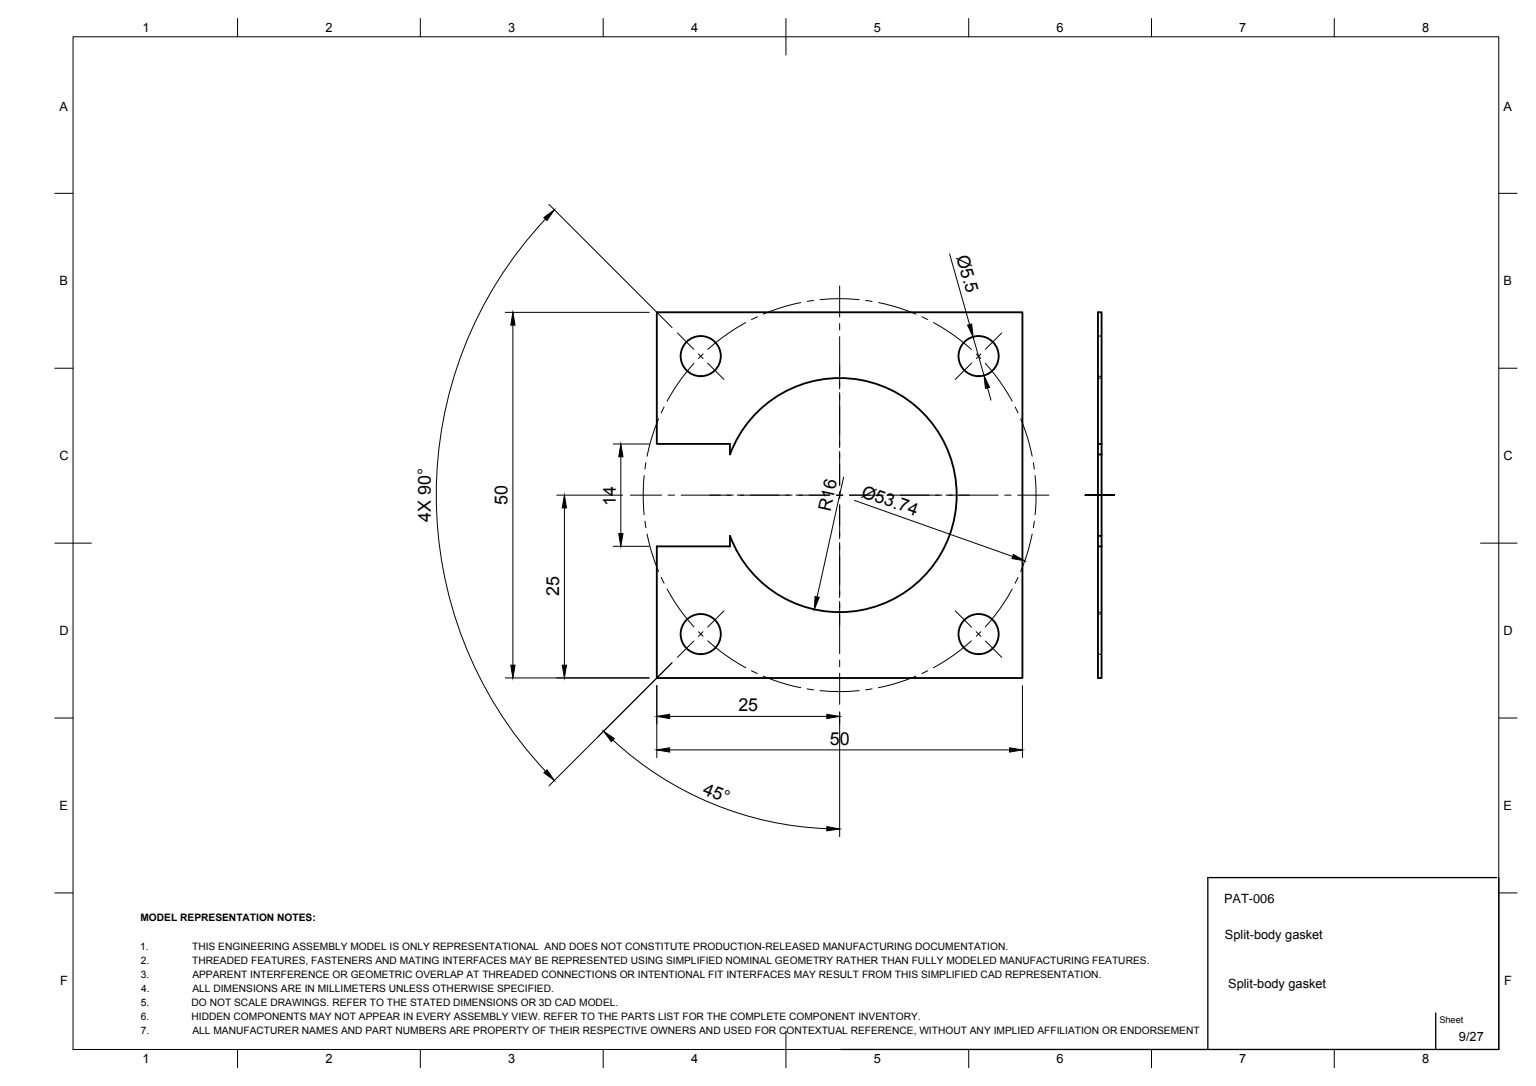
ISO-10303-21;
HEADER;
/* Generated by software containing ST-Developer
 * from STEP Tools, Inc. (www.steptools.com) 
 */

FILE_DESCRIPTION(
/* description */ ('Ball-type isolation valve (generic)'),
/* implementation_level */ '2;1');

FILE_NAME(
/* name */ 'Split-body gasket.step',
/* time_stamp */ '2026-10-27T10:53:05-07:00',
/* author */ (''),
/* organization */ (''),
/* preprocessor_version */ 'ST-DEVELOPER v20.2',
/* originating_system */ 'Autodesk Translation Framework v15.17.0.0',
/* authorisation */ '');

FILE_SCHEMA (('AUTOMOTIVE_DESIGN { 1 0 10303 214 3 1 1 }'));
ENDSEC;

DATA;
#10=MECHANICAL_DESIGN_GEOMETRIC_PRESENTATION_REPRESENTATION('',(#281),#7425);
#229=SHAPE_REPRESENTATION_RELATIONSHIP('SRR','None',#7539,#255);
#255=ADVANCED_BREP_SHAPE_REPRESENTATION('',(#307),#7402);
#281=STYLED_ITEM('',(#7723),#307);
#307=MANIFOLD_SOLID_BREP('Body1',#4086);
#365=FACE_BOUND('',#923,.T.);
#366=FACE_BOUND('',#924,.T.);
#367=FACE_BOUND('',#925,.T.);
#368=FACE_BOUND('',#926,.T.);
#369=FACE_BOUND('',#934,.T.);
#370=FACE_BOUND('',#935,.T.);
#371=FACE_BOUND('',#936,.T.);
#372=FACE_BOUND('',#937,.T.);
#445=PLANE('',#4521);
#446=PLANE('',#4522);
#447=PLANE('',#4523);
#448=PLANE('',#4524);
#449=PLANE('',#4525);
#450=PLANE('',#4527);
#451=PLANE('',#4528);
#452=PLANE('',#4531);
#453=PLANE('',#4532);
#454=PLANE('',#4533);
#455=PLANE('',#4534);
#631=FACE_OUTER_BOUND('',#914,.T.);
#632=FACE_OUTER_BOUND('',#915,.T.);
#633=FACE_OUTER_BOUND('',#916,.T.);
#634=FACE_OUTER_BOUND('',#917,.T.);
#635=FACE_OUTER_BOUND('',#918,.T.);
#636=FACE_OUTER_BOUND('',#919,.T.);
#637=FACE_OUTER_BOUND('',#920,.T.);
#638=FACE_OUTER_BOUND('',#921,.T.);
#639=FACE_OUTER_BOUND('',#922,.T.);
#640=FACE_OUTER_BOUND('',#927,.T.);
#641=FACE_OUTER_BOUND('',#928,.T.);
#642=FACE_OUTER_BOUND('',#929,.T.);
#643=FACE_OUTER_BOUND('',#930,.T.);
#644=FACE_OUTER_BOUND('',#931,.T.);
#645=FACE_OUTER_BOUND('',#932,.T.);
#646=FACE_OUTER_BOUND('',#933,.T.);
#914=EDGE_LOOP('',(#2987,#2988,#2989,#2990));
#915=EDGE_LOOP('',(#2991,#2992,#2993,#2994));
#916=EDGE_LOOP('',(#2995,#2996,#2997,#2998));
#917=EDGE_LOOP('',(#2999,#3000,#3001,#3002));
#918=EDGE_LOOP('',(#3003,#3004,#3005,#3006));
#919=EDGE_LOOP('',(#3007,#3008,#3009,#3010));
#920=EDGE_LOOP('',(#3011,#3012,#3013,#3014));
#921=EDGE_LOOP('',(#3015,#3016,#3017,#3018));
#922=EDGE_LOOP('',(#3019,#3020,#3021,#3022,#3023,#3024,#3025,#3026,#3027,
#3028));
#923=EDGE_LOOP('',(#3029));
#924=EDGE_LOOP('',(#3030));
#925=EDGE_LOOP('',(#3031));
#926=EDGE_LOOP('',(#3032));
#927=EDGE_LOOP('',(#3033,#3034,#3035,#3036));
#928=EDGE_LOOP('',(#3037,#3038,#3039,#3040));
#929=EDGE_LOOP('',(#3041,#3042,#3043,#3044));
#930=EDGE_LOOP('',(#3045,#3046,#3047,#3048));
#931=EDGE_LOOP('',(#3049,#3050,#3051,#3052));
#932=EDGE_LOOP('',(#3053,#3054,#3055,#3056));
#933=EDGE_LOOP('',(#3057,#3058,#3059,#3060,#3061,#3062,#3063,#3064,#3065,
#3066));
#934=EDGE_LOOP('',(#3067));
#935=EDGE_LOOP('',(#3068));
#936=EDGE_LOOP('',(#3069));
#937=EDGE_LOOP('',(#3070));
#1219=LINE('',#6441,#1527);
#1220=LINE('',#6447,#1528);
#1221=LINE('',#6453,#1529);
#1222=LINE('',#6459,#1530);
#1223=LINE('',#6464,#1531);
#1224=LINE('',#6466,#1532);
#1225=LINE('',#6468,#1533);
#1226=LINE('',#6469,#1534);
#1227=LINE('',#6473,#1535);
#1228=LINE('',#6475,#1536);
#1229=LINE('',#6477,#1537);
#1230=LINE('',#6478,#1538);
#1231=LINE('',#6481,#1539);
#1232=LINE('',#6483,#1540);
#1233=LINE('',#6484,#1541);
#1234=LINE('',#6487,#1542);
#1235=LINE('',#6489,#1543);
#1236=LINE('',#6490,#1544);
#1237=LINE('',#6494,#1545);
#1238=LINE('',#6496,#1546);
#1239=LINE('',#6498,#1547);
#1240=LINE('',#6500,#1548);
#1241=LINE('',#6501,#1549);
#1242=LINE('',#6504,#1550);
#1243=LINE('',#6505,#1551);
#1244=LINE('',#6508,#1552);
#1245=LINE('',#6509,#1553);
#1246=LINE('',#6514,#1554);
#1247=LINE('',#6515,#1555);
#1248=LINE('',#6518,#1556);
#1249=LINE('',#6519,#1557);
#1250=LINE('',#6521,#1558);
#1527=VECTOR('',#5176,0.275);
#1528=VECTOR('',#5183,0.275);
#1529=VECTOR('',#5190,0.275);
#1530=VECTOR('',#5197,0.275);
#1531=VECTOR('',#5202,1.);
#1532=VECTOR('',#5203,1.);
#1533=VECTOR('',#5204,1.);
#1534=VECTOR('',#5205,1.);
#1535=VECTOR('',#5208,1.);
#1536=VECTOR('',#5209,1.);
#1537=VECTOR('',#5210,1.);
#1538=VECTOR('',#5211,1.);
#1539=VECTOR('',#5214,1.);
#1540=VECTOR('',#5215,1.);
#1541=VECTOR('',#5216,1.);
#1542=VECTOR('',#5219,1.);
#1543=VECTOR('',#5220,1.);
#1544=VECTOR('',#5221,1.);
#1545=VECTOR('',#5226,1.);
#1546=VECTOR('',#5227,1.);
#1547=VECTOR('',#5228,1.);
#1548=VECTOR('',#5229,1.);
#1549=VECTOR('',#5230,1.);
#1550=VECTOR('',#5233,1.);
#1551=VECTOR('',#5234,1.);
#1552=VECTOR('',#5237,1.);
#1553=VECTOR('',#5238,1.);
#1554=VECTOR('',#5245,1.);
#1555=VECTOR('',#5246,1.);
#1556=VECTOR('',#5249,1.);
#1557=VECTOR('',#5250,1.);
#1558=VECTOR('',#5253,1.);
#1833=CIRCLE('',#4510,0.275);
#1834=CIRCLE('',#4511,0.275);
#1835=CIRCLE('',#4513,0.275);
#1836=CIRCLE('',#4514,0.275);
#1837=CIRCLE('',#4516,0.275);
#1838=CIRCLE('',#4517,0.275);
#1839=CIRCLE('',#4519,0.275);
#1840=CIRCLE('',#4520,0.275);
#1841=CIRCLE('',#4526,1.6);
#1842=CIRCLE('',#4530,1.6);
#2028=VERTEX_POINT('',#6438);
#2029=VERTEX_POINT('',#6440);
#2030=VERTEX_POINT('',#6444);
#2031=VERTEX_POINT('',#6446);
#2032=VERTEX_POINT('',#6450);
#2033=VERTEX_POINT('',#6452);
#2034=VERTEX_POINT('',#6456);
#2035=VERTEX_POINT('',#6458);
#2036=VERTEX_POINT('',#6462);
#2037=VERTEX_POINT('',#6463);
#2038=VERTEX_POINT('',#6465);
#2039=VERTEX_POINT('',#6467);
#2040=VERTEX_POINT('',#6471);
#2041=VERTEX_POINT('',#6472);
#2042=VERTEX_POINT('',#6474);
#2043=VERTEX_POINT('',#6476);
#2044=VERTEX_POINT('',#6480);
#2045=VERTEX_POINT('',#6482);
#2046=VERTEX_POINT('',#6486);
#2047=VERTEX_POINT('',#6488);
#2048=VERTEX_POINT('',#6493);
#2049=VERTEX_POINT('',#6495);
#2050=VERTEX_POINT('',#6497);
#2051=VERTEX_POINT('',#6499);
#2052=VERTEX_POINT('',#6503);
#2053=VERTEX_POINT('',#6507);
#2054=VERTEX_POINT('',#6513);
#2055=VERTEX_POINT('',#6517);
#2386=EDGE_CURVE('',#2028,#2028,#1833,.T.);
#2387=EDGE_CURVE('',#2028,#2029,#1219,.T.);
#2388=EDGE_CURVE('',#2029,#2029,#1834,.T.);
#2389=EDGE_CURVE('',#2030,#2030,#1835,.T.);
#2390=EDGE_CURVE('',#2030,#2031,#1220,.T.);
#2391=EDGE_CURVE('',#2031,#2031,#1836,.T.);
#2392=EDGE_CURVE('',#2032,#2032,#1837,.T.);
#2393=EDGE_CURVE('',#2032,#2033,#1221,.T.);
#2394=EDGE_CURVE('',#2033,#2033,#1838,.T.);
#2395=EDGE_CURVE('',#2034,#2034,#1839,.T.);
#2396=EDGE_CURVE('',#2034,#2035,#1222,.T.);
#2397=EDGE_CURVE('',#2035,#2035,#1840,.T.);
#2398=EDGE_CURVE('',#2036,#2037,#1223,.T.);
#2399=EDGE_CURVE('',#2036,#2038,#1224,.T.);
#2400=EDGE_CURVE('',#2039,#2038,#1225,.T.);
#2401=EDGE_CURVE('',#2037,#2039,#1226,.T.);
#2402=EDGE_CURVE('',#2040,#2041,#1227,.T.);
#2403=EDGE_CURVE('',#2040,#2042,#1228,.T.);
#2404=EDGE_CURVE('',#2043,#2042,#1229,.T.);
#2405=EDGE_CURVE('',#2041,#2043,#1230,.T.);
#2406=EDGE_CURVE('',#2044,#2036,#1231,.T.);
#2407=EDGE_CURVE('',#2045,#2044,#1232,.T.);
#2408=EDGE_CURVE('',#2038,#2045,#1233,.T.);
#2409=EDGE_CURVE('',#2046,#2040,#1234,.T.);
#2410=EDGE_CURVE('',#2047,#2046,#1235,.T.);
#2411=EDGE_CURVE('',#2042,#2047,#1236,.T.);
#2412=EDGE_CURVE('',#2045,#2043,#1841,.T.);
#2413=EDGE_CURVE('',#2047,#2048,#1237,.T.);
#2414=EDGE_CURVE('',#2048,#2049,#1238,.T.);
#2415=EDGE_CURVE('',#2049,#2050,#1239,.T.);
#2416=EDGE_CURVE('',#2050,#2051,#1240,.T.);
#2417=EDGE_CURVE('',#2051,#2039,#1241,.T.);
#2418=EDGE_CURVE('',#2052,#2046,#1242,.T.);
#2419=EDGE_CURVE('',#2052,#2048,#1243,.T.);
#2420=EDGE_CURVE('',#2053,#2051,#1244,.T.);
#2421=EDGE_CURVE('',#2037,#2053,#1245,.T.);
#2422=EDGE_CURVE('',#2041,#2044,#1842,.T.);
#2423=EDGE_CURVE('',#2053,#2054,#1246,.T.);
#2424=EDGE_CURVE('',#2054,#2050,#1247,.T.);
#2425=EDGE_CURVE('',#2054,#2055,#1248,.T.);
#2426=EDGE_CURVE('',#2055,#2049,#1249,.T.);
#2427=EDGE_CURVE('',#2055,#2052,#1250,.T.);
#2987=ORIENTED_EDGE('',*,*,#2386,.F.);
#2988=ORIENTED_EDGE('',*,*,#2387,.T.);
#2989=ORIENTED_EDGE('',*,*,#2388,.F.);
#2990=ORIENTED_EDGE('',*,*,#2387,.F.);
#2991=ORIENTED_EDGE('',*,*,#2389,.F.);
#2992=ORIENTED_EDGE('',*,*,#2390,.T.);
#2993=ORIENTED_EDGE('',*,*,#2391,.F.);
#2994=ORIENTED_EDGE('',*,*,#2390,.F.);
#2995=ORIENTED_EDGE('',*,*,#2392,.F.);
#2996=ORIENTED_EDGE('',*,*,#2393,.T.);
#2997=ORIENTED_EDGE('',*,*,#2394,.F.);
#2998=ORIENTED_EDGE('',*,*,#2393,.F.);
#2999=ORIENTED_EDGE('',*,*,#2395,.F.);
#3000=ORIENTED_EDGE('',*,*,#2396,.T.);
#3001=ORIENTED_EDGE('',*,*,#2397,.F.);
#3002=ORIENTED_EDGE('',*,*,#2396,.F.);
#3003=ORIENTED_EDGE('',*,*,#2398,.F.);
#3004=ORIENTED_EDGE('',*,*,#2399,.T.);
#3005=ORIENTED_EDGE('',*,*,#2400,.F.);
#3006=ORIENTED_EDGE('',*,*,#2401,.F.);
#3007=ORIENTED_EDGE('',*,*,#2402,.F.);
#3008=ORIENTED_EDGE('',*,*,#2403,.T.);
#3009=ORIENTED_EDGE('',*,*,#2404,.F.);
#3010=ORIENTED_EDGE('',*,*,#2405,.F.);
#3011=ORIENTED_EDGE('',*,*,#2406,.F.);
#3012=ORIENTED_EDGE('',*,*,#2407,.F.);
#3013=ORIENTED_EDGE('',*,*,#2408,.F.);
#3014=ORIENTED_EDGE('',*,*,#2399,.F.);
#3015=ORIENTED_EDGE('',*,*,#2409,.F.);
#3016=ORIENTED_EDGE('',*,*,#2410,.F.);
#3017=ORIENTED_EDGE('',*,*,#2411,.F.);
#3018=ORIENTED_EDGE('',*,*,#2403,.F.);
#3019=ORIENTED_EDGE('',*,*,#2400,.T.);
#3020=ORIENTED_EDGE('',*,*,#2408,.T.);
#3021=ORIENTED_EDGE('',*,*,#2412,.T.);
#3022=ORIENTED_EDGE('',*,*,#2404,.T.);
#3023=ORIENTED_EDGE('',*,*,#2411,.T.);
#3024=ORIENTED_EDGE('',*,*,#2413,.T.);
#3025=ORIENTED_EDGE('',*,*,#2414,.T.);
#3026=ORIENTED_EDGE('',*,*,#2415,.T.);
#3027=ORIENTED_EDGE('',*,*,#2416,.T.);
#3028=ORIENTED_EDGE('',*,*,#2417,.T.);
#3029=ORIENTED_EDGE('',*,*,#2388,.T.);
#3030=ORIENTED_EDGE('',*,*,#2391,.T.);
#3031=ORIENTED_EDGE('',*,*,#2394,.T.);
#3032=ORIENTED_EDGE('',*,*,#2397,.T.);
#3033=ORIENTED_EDGE('',*,*,#2410,.T.);
#3034=ORIENTED_EDGE('',*,*,#2418,.F.);
#3035=ORIENTED_EDGE('',*,*,#2419,.T.);
#3036=ORIENTED_EDGE('',*,*,#2413,.F.);
#3037=ORIENTED_EDGE('',*,*,#2401,.T.);
#3038=ORIENTED_EDGE('',*,*,#2417,.F.);
#3039=ORIENTED_EDGE('',*,*,#2420,.F.);
#3040=ORIENTED_EDGE('',*,*,#2421,.F.);
#3041=ORIENTED_EDGE('',*,*,#2407,.T.);
#3042=ORIENTED_EDGE('',*,*,#2422,.F.);
#3043=ORIENTED_EDGE('',*,*,#2405,.T.);
#3044=ORIENTED_EDGE('',*,*,#2412,.F.);
#3045=ORIENTED_EDGE('',*,*,#2423,.F.);
#3046=ORIENTED_EDGE('',*,*,#2420,.T.);
#3047=ORIENTED_EDGE('',*,*,#2416,.F.);
#3048=ORIENTED_EDGE('',*,*,#2424,.F.);
#3049=ORIENTED_EDGE('',*,*,#2425,.F.);
#3050=ORIENTED_EDGE('',*,*,#2424,.T.);
#3051=ORIENTED_EDGE('',*,*,#2415,.F.);
#3052=ORIENTED_EDGE('',*,*,#2426,.F.);
#3053=ORIENTED_EDGE('',*,*,#2427,.F.);
#3054=ORIENTED_EDGE('',*,*,#2426,.T.);
#3055=ORIENTED_EDGE('',*,*,#2414,.F.);
#3056=ORIENTED_EDGE('',*,*,#2419,.F.);
#3057=ORIENTED_EDGE('',*,*,#2398,.T.);
#3058=ORIENTED_EDGE('',*,*,#2421,.T.);
#3059=ORIENTED_EDGE('',*,*,#2423,.T.);
#3060=ORIENTED_EDGE('',*,*,#2425,.T.);
#3061=ORIENTED_EDGE('',*,*,#2427,.T.);
#3062=ORIENTED_EDGE('',*,*,#2418,.T.);
#3063=ORIENTED_EDGE('',*,*,#2409,.T.);
#3064=ORIENTED_EDGE('',*,*,#2402,.T.);
#3065=ORIENTED_EDGE('',*,*,#2422,.T.);
#3066=ORIENTED_EDGE('',*,*,#2406,.T.);
#3067=ORIENTED_EDGE('',*,*,#2386,.T.);
#3068=ORIENTED_EDGE('',*,*,#2389,.T.);
#3069=ORIENTED_EDGE('',*,*,#2392,.T.);
#3070=ORIENTED_EDGE('',*,*,#2395,.T.);
#3787=CYLINDRICAL_SURFACE('',#4509,0.275);
#3788=CYLINDRICAL_SURFACE('',#4512,0.275);
#3789=CYLINDRICAL_SURFACE('',#4515,0.275);
#3790=CYLINDRICAL_SURFACE('',#4518,0.275);
#3791=CYLINDRICAL_SURFACE('',#4529,1.6);
#3885=ADVANCED_FACE('',(#631),#3787,.F.);
#3886=ADVANCED_FACE('',(#632),#3788,.F.);
#3887=ADVANCED_FACE('',(#633),#3789,.F.);
#3888=ADVANCED_FACE('',(#634),#3790,.F.);
#3889=ADVANCED_FACE('',(#635),#445,.F.);
#3890=ADVANCED_FACE('',(#636),#446,.F.);
#3891=ADVANCED_FACE('',(#637),#447,.F.);
#3892=ADVANCED_FACE('',(#638),#448,.F.);
#3893=ADVANCED_FACE('',(#639,#365,#366,#367,#368),#449,.T.);
#3894=ADVANCED_FACE('',(#640),#450,.T.);
#3895=ADVANCED_FACE('',(#641),#451,.T.);
#3896=ADVANCED_FACE('',(#642),#3791,.F.);
#3897=ADVANCED_FACE('',(#643),#452,.T.);
#3898=ADVANCED_FACE('',(#644),#453,.T.);
#3899=ADVANCED_FACE('',(#645),#454,.T.);
#3900=ADVANCED_FACE('',(#646,#369,#370,#371,#372),#455,.F.);
#4086=CLOSED_SHELL('',(#3885,#3886,#3887,#3888,#3889,#3890,#3891,#3892,
#3893,#3894,#3895,#3896,#3897,#3898,#3899,#3900));
#4508=AXIS2_PLACEMENT_3D('',#6436,#5170,#5171);
#4509=AXIS2_PLACEMENT_3D('',#6437,#5172,#5173);
#4510=AXIS2_PLACEMENT_3D('',#6439,#5174,#5175);
#4511=AXIS2_PLACEMENT_3D('',#6442,#5177,#5178);
#4512=AXIS2_PLACEMENT_3D('',#6443,#5179,#5180);
#4513=AXIS2_PLACEMENT_3D('',#6445,#5181,#5182);
#4514=AXIS2_PLACEMENT_3D('',#6448,#5184,#5185);
#4515=AXIS2_PLACEMENT_3D('',#6449,#5186,#5187);
#4516=AXIS2_PLACEMENT_3D('',#6451,#5188,#5189);
#4517=AXIS2_PLACEMENT_3D('',#6454,#5191,#5192);
#4518=AXIS2_PLACEMENT_3D('',#6455,#5193,#5194);
#4519=AXIS2_PLACEMENT_3D('',#6457,#5195,#5196);
#4520=AXIS2_PLACEMENT_3D('',#6460,#5198,#5199);
#4521=AXIS2_PLACEMENT_3D('',#6461,#5200,#5201);
#4522=AXIS2_PLACEMENT_3D('',#6470,#5206,#5207);
#4523=AXIS2_PLACEMENT_3D('',#6479,#5212,#5213);
#4524=AXIS2_PLACEMENT_3D('',#6485,#5217,#5218);
#4525=AXIS2_PLACEMENT_3D('',#6491,#5222,#5223);
#4526=AXIS2_PLACEMENT_3D('',#6492,#5224,#5225);
#4527=AXIS2_PLACEMENT_3D('',#6502,#5231,#5232);
#4528=AXIS2_PLACEMENT_3D('',#6506,#5235,#5236);
#4529=AXIS2_PLACEMENT_3D('',#6510,#5239,#5240);
#4530=AXIS2_PLACEMENT_3D('',#6511,#5241,#5242);
#4531=AXIS2_PLACEMENT_3D('',#6512,#5243,#5244);
#4532=AXIS2_PLACEMENT_3D('',#6516,#5247,#5248);
#4533=AXIS2_PLACEMENT_3D('',#6520,#5251,#5252);
#4534=AXIS2_PLACEMENT_3D('',#6522,#5254,#5255);
#5170=DIRECTION('axis',(0.,0.,1.));
#5171=DIRECTION('refdir',(1.,0.,0.));
#5172=DIRECTION('center_axis',(0.,1.,0.));
#5173=DIRECTION('ref_axis',(1.,0.,0.));
#5174=DIRECTION('center_axis',(0.,1.,0.));
#5175=DIRECTION('ref_axis',(1.,0.,0.));
#5176=DIRECTION('',(0.,1.,0.));
#5177=DIRECTION('center_axis',(0.,-1.,0.));
#5178=DIRECTION('ref_axis',(1.,0.,0.));
#5179=DIRECTION('center_axis',(0.,1.,0.));
#5180=DIRECTION('ref_axis',(1.,0.,0.));
#5181=DIRECTION('center_axis',(0.,1.,0.));
#5182=DIRECTION('ref_axis',(1.,0.,0.));
#5183=DIRECTION('',(0.,1.,0.));
#5184=DIRECTION('center_axis',(0.,-1.,0.));
#5185=DIRECTION('ref_axis',(1.,0.,0.));
#5186=DIRECTION('center_axis',(0.,1.,0.));
#5187=DIRECTION('ref_axis',(1.,0.,0.));
#5188=DIRECTION('center_axis',(0.,1.,0.));
#5189=DIRECTION('ref_axis',(1.,0.,0.));
#5190=DIRECTION('',(0.,1.,0.));
#5191=DIRECTION('center_axis',(0.,-1.,0.));
#5192=DIRECTION('ref_axis',(1.,0.,0.));
#5193=DIRECTION('center_axis',(0.,1.,0.));
#5194=DIRECTION('ref_axis',(1.,0.,0.));
#5195=DIRECTION('center_axis',(0.,1.,0.));
#5196=DIRECTION('ref_axis',(1.,0.,0.));
#5197=DIRECTION('',(0.,1.,0.));
#5198=DIRECTION('center_axis',(0.,-1.,0.));
#5199=DIRECTION('ref_axis',(1.,0.,0.));
#5200=DIRECTION('center_axis',(-1.,0.,0.));
#5201=DIRECTION('ref_axis',(0.,0.,1.));
#5202=DIRECTION('',(0.,0.,1.));
#5203=DIRECTION('',(0.,1.,0.));
#5204=DIRECTION('',(0.,0.,-1.));
#5205=DIRECTION('',(0.,1.,0.));
#5206=DIRECTION('center_axis',(0.,0.,-1.));
#5207=DIRECTION('ref_axis',(-1.,0.,0.));
#5208=DIRECTION('',(-1.,0.,0.));
#5209=DIRECTION('',(0.,1.,0.));
#5210=DIRECTION('',(1.,0.,0.));
#5211=DIRECTION('',(0.,1.,0.));
#5212=DIRECTION('center_axis',(0.,0.,-1.));
#5213=DIRECTION('ref_axis',(-1.,0.,0.));
#5214=DIRECTION('',(-1.,0.,0.));
#5215=DIRECTION('',(0.,-1.,0.));
#5216=DIRECTION('',(1.,0.,0.));
#5217=DIRECTION('center_axis',(1.,0.,0.));
#5218=DIRECTION('ref_axis',(0.,0.,-1.));
#5219=DIRECTION('',(0.,0.,-1.));
#5220=DIRECTION('',(0.,-1.,0.));
#5221=DIRECTION('',(0.,0.,1.));
#5222=DIRECTION('center_axis',(0.,1.,0.));
#5223=DIRECTION('ref_axis',(0.,0.,1.));
#5224=DIRECTION('center_axis',(0.,-1.,0.));
#5225=DIRECTION('ref_axis',(1.,0.,0.));
#5226=DIRECTION('',(1.,0.,0.));
#5227=DIRECTION('',(0.,0.,-1.));
#5228=DIRECTION('',(-1.,0.,0.));
#5229=DIRECTION('',(0.,0.,1.));
#5230=DIRECTION('',(1.,0.,0.));
#5231=DIRECTION('center_axis',(0.,0.,1.));
#5232=DIRECTION('ref_axis',(1.,0.,0.));
#5233=DIRECTION('',(-1.,0.,0.));
#5234=DIRECTION('',(0.,1.,0.));
#5235=DIRECTION('center_axis',(0.,0.,1.));
#5236=DIRECTION('ref_axis',(1.,0.,0.));
#5237=DIRECTION('',(0.,1.,0.));
#5238=DIRECTION('',(-1.,0.,0.));
#5239=DIRECTION('center_axis',(0.,1.,0.));
#5240=DIRECTION('ref_axis',(-1.83697019872103E-16,0.,-1.));
#5241=DIRECTION('center_axis',(0.,1.,0.));
#5242=DIRECTION('ref_axis',(1.,0.,0.));
#5243=DIRECTION('center_axis',(-1.,0.,0.));
#5244=DIRECTION('ref_axis',(0.,0.,1.));
#5245=DIRECTION('',(0.,0.,-1.));
#5246=DIRECTION('',(0.,1.,0.));
#5247=DIRECTION('center_axis',(0.,0.,-1.));
#5248=DIRECTION('ref_axis',(-1.,0.,0.));
#5249=DIRECTION('',(1.,0.,0.));
#5250=DIRECTION('',(0.,1.,0.));
#5251=DIRECTION('center_axis',(1.,0.,0.));
#5252=DIRECTION('ref_axis',(0.,0.,-1.));
#5253=DIRECTION('',(0.,0.,1.));
#5254=DIRECTION('center_axis',(0.,1.,0.));
#5255=DIRECTION('ref_axis',(1.,0.,0.));
#6436=CARTESIAN_POINT('',(0.,0.,0.));
#6437=CARTESIAN_POINT('Origin',(1.9,-0.1,3.1));
#6438=CARTESIAN_POINT('',(1.625,-0.025,3.1));
#6439=CARTESIAN_POINT('Origin',(1.9,-0.025,3.1));
#6440=CARTESIAN_POINT('',(1.625,0.025,3.1));
#6441=CARTESIAN_POINT('',(1.625,-0.1,3.1));
#6442=CARTESIAN_POINT('Origin',(1.9,0.025,3.1));
#6443=CARTESIAN_POINT('Origin',(-1.9,-0.1,6.9));
#6444=CARTESIAN_POINT('',(-2.175,-0.025,6.9));
#6445=CARTESIAN_POINT('Origin',(-1.9,-0.025,6.9));
#6446=CARTESIAN_POINT('',(-2.175,0.025,6.9));
#6447=CARTESIAN_POINT('',(-2.175,-0.1,6.9));
#6448=CARTESIAN_POINT('Origin',(-1.9,0.025,6.9));
#6449=CARTESIAN_POINT('Origin',(-1.9,-0.1,3.1));
#6450=CARTESIAN_POINT('',(-2.175,-0.025,3.1));
#6451=CARTESIAN_POINT('Origin',(-1.9,-0.025,3.1));
#6452=CARTESIAN_POINT('',(-2.175,0.025,3.1));
#6453=CARTESIAN_POINT('',(-2.175,-0.1,3.1));
#6454=CARTESIAN_POINT('Origin',(-1.9,0.025,3.1));
#6455=CARTESIAN_POINT('Origin',(1.9,-0.1,6.9));
#6456=CARTESIAN_POINT('',(1.625,-0.025,6.9));
#6457=CARTESIAN_POINT('Origin',(1.9,-0.025,6.9));
#6458=CARTESIAN_POINT('',(1.625,0.025,6.9));
#6459=CARTESIAN_POINT('',(1.625,-0.1,6.9));
#6460=CARTESIAN_POINT('Origin',(1.9,0.025,6.9));
#6461=CARTESIAN_POINT('Origin',(-0.7,-0.1,6.5));
#6462=CARTESIAN_POINT('',(-0.7,-0.025,6.5));
#6463=CARTESIAN_POINT('',(-0.7,-0.025,7.5));
#6464=CARTESIAN_POINT('',(-0.7,-0.025,5.75));
#6465=CARTESIAN_POINT('',(-0.7,0.025,6.5));
#6466=CARTESIAN_POINT('',(-0.7,-0.1,6.5));
#6467=CARTESIAN_POINT('',(-0.7,0.025,7.5));
#6468=CARTESIAN_POINT('',(-0.7,0.025,5.75));
#6469=CARTESIAN_POINT('',(-0.7,-0.0625,7.5));
#6470=CARTESIAN_POINT('Origin',(0.7,-0.1,6.5));
#6471=CARTESIAN_POINT('',(0.7,-0.025,6.5));
#6472=CARTESIAN_POINT('',(0.556776436283003,-0.025,6.5));
#6473=CARTESIAN_POINT('',(0.35,-0.025,6.5));
#6474=CARTESIAN_POINT('',(0.7,0.025,6.5));
#6475=CARTESIAN_POINT('',(0.7,-0.1,6.5));
#6476=CARTESIAN_POINT('',(0.556776436283003,0.025,6.5));
#6477=CARTESIAN_POINT('',(0.35,0.025,6.5));
#6478=CARTESIAN_POINT('',(0.556776436283003,-0.1,6.5));
#6479=CARTESIAN_POINT('Origin',(0.7,-0.1,6.5));
#6480=CARTESIAN_POINT('',(-0.556776436283003,-0.025,6.5));
#6481=CARTESIAN_POINT('',(0.35,-0.025,6.5));
#6482=CARTESIAN_POINT('',(-0.556776436283003,0.025,6.5));
#6483=CARTESIAN_POINT('',(-0.556776436283003,-0.1,6.5));
#6484=CARTESIAN_POINT('',(0.35,0.025,6.5));
#6485=CARTESIAN_POINT('Origin',(0.7,-0.1,7.6));
#6486=CARTESIAN_POINT('',(0.7,-0.025,7.5));
#6487=CARTESIAN_POINT('',(0.7,-0.025,6.3));
#6488=CARTESIAN_POINT('',(0.7,0.025,7.5));
#6489=CARTESIAN_POINT('',(0.7,-0.0625,7.5));
#6490=CARTESIAN_POINT('',(0.7,0.025,6.3));
#6491=CARTESIAN_POINT('Origin',(0.,0.025,5.));
#6492=CARTESIAN_POINT('Origin',(0.,0.025,5.));
#6493=CARTESIAN_POINT('',(2.5,0.025,7.5));
#6494=CARTESIAN_POINT('',(2.5,0.025,7.5));
#6495=CARTESIAN_POINT('',(2.5,0.025,2.5));
#6496=CARTESIAN_POINT('',(2.5,0.025,2.5));
#6497=CARTESIAN_POINT('',(-2.5,0.025,2.5));
#6498=CARTESIAN_POINT('',(-2.5,0.025,2.5));
#6499=CARTESIAN_POINT('',(-2.5,0.025,7.5));
#6500=CARTESIAN_POINT('',(-2.5,0.025,7.5));
#6501=CARTESIAN_POINT('',(2.5,0.025,7.5));
#6502=CARTESIAN_POINT('Origin',(-2.5,-0.025,7.5));
#6503=CARTESIAN_POINT('',(2.5,-0.025,7.5));
#6504=CARTESIAN_POINT('',(2.5,-0.025,7.5));
#6505=CARTESIAN_POINT('',(2.5,-0.025,7.5));
#6506=CARTESIAN_POINT('Origin',(-2.5,-0.025,7.5));
#6507=CARTESIAN_POINT('',(-2.5,-0.025,7.5));
#6508=CARTESIAN_POINT('',(-2.5,-0.025,7.5));
#6509=CARTESIAN_POINT('',(2.5,-0.025,7.5));
#6510=CARTESIAN_POINT('Origin',(0.,-0.1,5.));
#6511=CARTESIAN_POINT('Origin',(0.,-0.025,5.));
#6512=CARTESIAN_POINT('Origin',(-2.5,-0.025,2.5));
#6513=CARTESIAN_POINT('',(-2.5,-0.025,2.5));
#6514=CARTESIAN_POINT('',(-2.5,-0.025,7.5));
#6515=CARTESIAN_POINT('',(-2.5,-0.025,2.5));
#6516=CARTESIAN_POINT('Origin',(2.5,-0.025,2.5));
#6517=CARTESIAN_POINT('',(2.5,-0.025,2.5));
#6518=CARTESIAN_POINT('',(-2.5,-0.025,2.5));
#6519=CARTESIAN_POINT('',(2.5,-0.025,2.5));
#6520=CARTESIAN_POINT('Origin',(2.5,-0.025,7.5));
#6521=CARTESIAN_POINT('',(2.5,-0.025,2.5));
#6522=CARTESIAN_POINT('Origin',(0.,-0.025,5.));
#7372=UNCERTAINTY_MEASURE_WITH_UNIT(LENGTH_MEASURE(0.001),#7426,
'DISTANCE_ACCURACY_VALUE',
'Maximum model space distance between geometric entities at asserted c
onnectivities');
#7395=UNCERTAINTY_MEASURE_WITH_UNIT(LENGTH_MEASURE(0.001),#7426,
'DISTANCE_ACCURACY_VALUE',
'Maximum model space distance between geometric entities at asserted c
onnectivities');
#7402=(
GEOMETRIC_REPRESENTATION_CONTEXT(3)
GLOBAL_UNCERTAINTY_ASSIGNED_CONTEXT((#7372))
GLOBAL_UNIT_ASSIGNED_CONTEXT((#7426,#7428,#7429))
REPRESENTATION_CONTEXT('','3D')
);
#7425=(
GEOMETRIC_REPRESENTATION_CONTEXT(3)
GLOBAL_UNCERTAINTY_ASSIGNED_CONTEXT((#7395))
GLOBAL_UNIT_ASSIGNED_CONTEXT((#7426,#7428,#7429))
REPRESENTATION_CONTEXT('','3D')
);
#7426=(
LENGTH_UNIT()
NAMED_UNIT(*)
SI_UNIT(.CENTI.,.METRE.)
);
#7428=(
NAMED_UNIT(*)
PLANE_ANGLE_UNIT()
SI_UNIT($,.RADIAN.)
);
#7429=(
NAMED_UNIT(*)
SI_UNIT($,.STERADIAN.)
SOLID_ANGLE_UNIT()
);
#7436=SHAPE_DEFINITION_REPRESENTATION(#7465,#7539);
#7465=PRODUCT_DEFINITION_SHAPE('',$,#7569);
#7539=SHAPE_REPRESENTATION('',(#4508),#7402);
#7562=PRODUCT_DEFINITION_CONTEXT('part definition',#7651,'design');
#7569=PRODUCT_DEFINITION('Split-body gasket','Split-body gasket',#7598,
#7562);
#7598=PRODUCT_DEFINITION_FORMATION('',$,#7659);
#7651=APPLICATION_CONTEXT(
'Core Data for Automotive Mechanical Design Process');
#7652=PRODUCT_CONTEXT('part definition',#7651,'mechanical');
#7659=PRODUCT('Split-body gasket','Split-body gasket',
'Split-body gasket',(#7652));
#7717=COLOUR_RGB('Dark Blue',0.08,0.2,0.34);
#7718=FILL_AREA_STYLE_COLOUR('',#7717);
#7719=FILL_AREA_STYLE('',(#7718));
#7720=SURFACE_STYLE_FILL_AREA(#7719);
#7721=SURFACE_SIDE_STYLE('',(#7720));
#7722=SURFACE_STYLE_USAGE(.BOTH.,#7721);
#7723=PRESENTATION_STYLE_ASSIGNMENT((#7722));
ENDSEC;
END-ISO-10303-21;
